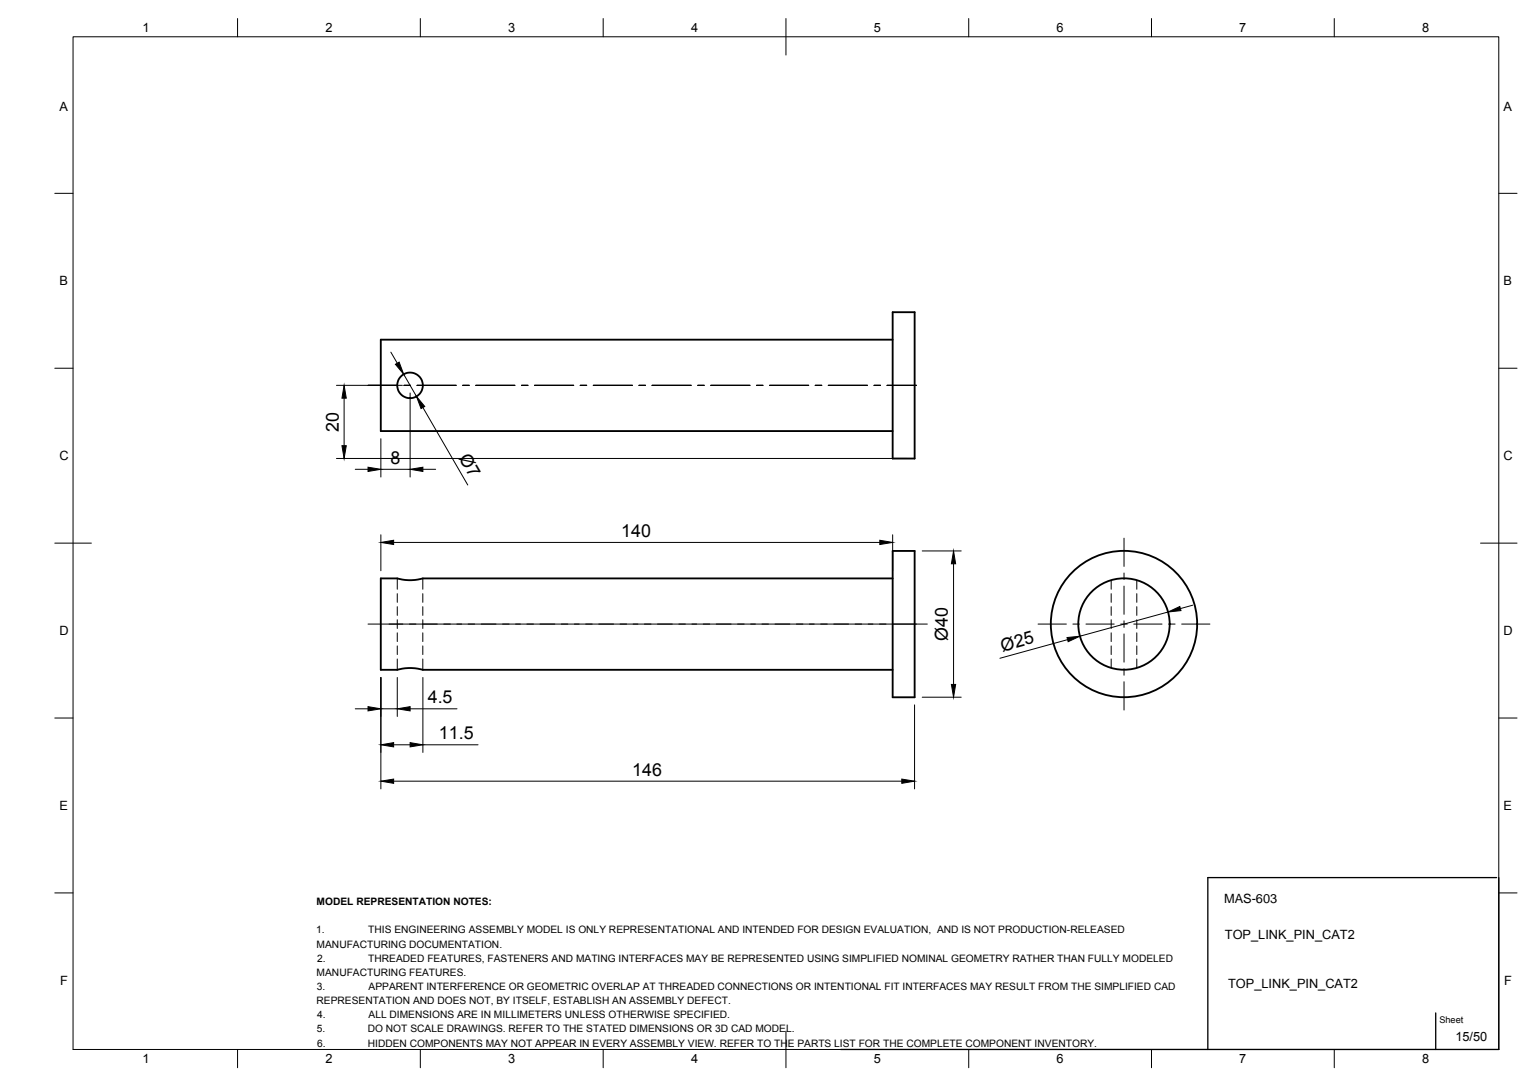
ISO-10303-21;
HEADER;
FILE_DESCRIPTION((''),'2;1');
FILE_NAME('TOP_LINK_PIN_CAT2.step','2026-10-01T22:06:14-07:00',(''),(''),'','','');
FILE_SCHEMA (('AUTOMOTIVE_DESIGN { 1 0 10303 214 3 1 1 }'));
ENDSEC;
DATA;
#10=MECHANICAL_DESIGN_GEOMETRIC_PRESENTATION_REPRESENTATION('',(#989),#50440);
#15=B_SPLINE_CURVE_WITH_KNOTS('',3,(#44967,#44968,#44969,#44970,#44971,
#44972,#44973,#44974,#44975,#44976,#44977,#44978,#44979,#44980,#44981,#44982,
#44983,#44984),.UNSPECIFIED.,.F.,.F.,(4,2,2,2,2,2,2,2,4),(0.,0.132623145855944,
0.265246291711889,0.39783980012189,0.530433308531892,0.663026816941894,
0.795620325351895,0.92824347120784,1.06086661706378),.UNSPECIFIED.) ;
#16=B_SPLINE_CURVE_WITH_KNOTS('',3,(#44985,#44986,#44987,#44988,#44989,
#44990,#44991,#44992,#44993,#44994,#44995,#44996,#44997,#44998,#44999,#45000,
#45001,#45002),.UNSPECIFIED.,.F.,.F.,(4,2,2,2,2,2,2,2,4),(1.06086661706378,
1.19348976291973,1.32611290877567,1.45870641718567,1.59129992559568,1.72389343400568,
1.85648694241568,1.98911008827162,2.12173323412757),.UNSPECIFIED.) ;
#17=B_SPLINE_CURVE_WITH_KNOTS('',3,(#45006,#45007,#45008,#45009,#45010,
#45011,#45012,#45013,#45014,#45015,#45016,#45017,#45018,#45019,#45020,#45021,
#45022,#45023),.UNSPECIFIED.,.F.,.F.,(4,2,2,2,2,2,2,2,4),(0.,0.132623145855943,
0.265246291711887,0.397839800121889,0.530433308531891,0.663026816941892,
0.795620325351894,0.928243471207838,1.06086661706378),.UNSPECIFIED.) ;
#18=B_SPLINE_CURVE_WITH_KNOTS('',3,(#45024,#45025,#45026,#45027,#45028,
#45029,#45030,#45031,#45032,#45033,#45034,#45035,#45036,#45037,#45038,#45039,
#45040,#45041),.UNSPECIFIED.,.F.,.F.,(4,2,2,2,2,2,2,2,4),(1.06086661706378,
1.19348976291973,1.32611290877567,1.45870641718567,1.59129992559567,1.72389343400568,
1.85648694241568,1.98911008827162,2.12173323412757),.UNSPECIFIED.) ;
#899=SHAPE_REPRESENTATION_RELATIONSHIP('SRR','None',#50630,#944) ;
#944=ADVANCED_BREP_SHAPE_REPRESENTATION('',(#1044),#50399) ;
#989=STYLED_ITEM('',(#50883),#1044) ;
#1044=MANIFOLD_SOLID_BREP('TOP_LINK_PIN_CAT2',#28656) ;
#1273=FACE_BOUND('',#4736,.T.) ;
#1274=FACE_BOUND('',#4740,.T.) ;
#1275=FACE_BOUND('',#4741,.T.) ;
#1929=PLANE('',#30266) ;
#1930=PLANE('',#30271) ;
#1931=PLANE('',#30274) ;
#3019=FACE_OUTER_BOUND('',#4734,.T.) ;
#3020=FACE_OUTER_BOUND('',#4735,.T.) ;
#3021=FACE_OUTER_BOUND('',#4737,.T.) ;
#3022=FACE_OUTER_BOUND('',#4738,.T.) ;
#3023=FACE_OUTER_BOUND('',#4739,.T.) ;
#3024=FACE_OUTER_BOUND('',#4742,.T.) ;
#4734=EDGE_LOOP('',(#22133,#22134,#22135,#22136,#22137,#22138)) ;
#4735=EDGE_LOOP('',(#22139)) ;
#4736=EDGE_LOOP('',(#22140)) ;
#4737=EDGE_LOOP('',(#22141,#22142,#22143,#22144)) ;
#4738=EDGE_LOOP('',(#22145)) ;
#4739=EDGE_LOOP('',(#22146,#22147,#22148,#22149)) ;
#4740=EDGE_LOOP('',(#22150,#22151)) ;
#4741=EDGE_LOOP('',(#22152,#22153)) ;
#4742=EDGE_LOOP('',(#22154)) ;
#7138=LINE('',#45004,#9610) ;
#7139=LINE('',#45049,#9611) ;
#7140=LINE('',#45055,#9612) ;
#9610=VECTOR('',#35895,0.35) ;
#9611=VECTOR('',#35904,2.) ;
#9612=VECTOR('',#35913,1.25) ;
#11002=CIRCLE('',#30267,2.) ;
#11003=CIRCLE('',#30268,1.25) ;
#11004=CIRCLE('',#30270,2.) ;
#11005=CIRCLE('',#30273,1.25) ;
#13028=VERTEX_POINT('',#44965) ;
#13029=VERTEX_POINT('',#44966) ;
#13030=VERTEX_POINT('',#45003) ;
#13031=VERTEX_POINT('',#45005) ;
#13032=VERTEX_POINT('',#45043) ;
#13033=VERTEX_POINT('',#45045) ;
#13034=VERTEX_POINT('',#45048) ;
#13035=VERTEX_POINT('',#45053) ;
#16332=EDGE_CURVE('',#13028,#13029,#15,.T.) ;
#16333=EDGE_CURVE('',#13029,#13028,#16,.T.) ;
#16334=EDGE_CURVE('',#13029,#13030,#7138,.T.) ;
#16335=EDGE_CURVE('',#13031,#13030,#17,.T.) ;
#16336=EDGE_CURVE('',#13030,#13031,#18,.T.) ;
#16337=EDGE_CURVE('',#13032,#13032,#11002,.T.) ;
#16338=EDGE_CURVE('',#13033,#13033,#11003,.T.) ;
#16339=EDGE_CURVE('',#13032,#13034,#7139,.T.) ;
#16340=EDGE_CURVE('',#13034,#13034,#11004,.T.) ;
#16341=EDGE_CURVE('',#13035,#13035,#11005,.T.) ;
#16342=EDGE_CURVE('',#13035,#13033,#7140,.T.) ;
#22133=ORIENTED_EDGE('',*,*,#16332,.F.) ;
#22134=ORIENTED_EDGE('',*,*,#16333,.F.) ;
#22135=ORIENTED_EDGE('',*,*,#16334,.T.) ;
#22136=ORIENTED_EDGE('',*,*,#16335,.F.) ;
#22137=ORIENTED_EDGE('',*,*,#16336,.F.) ;
#22138=ORIENTED_EDGE('',*,*,#16334,.F.) ;
#22139=ORIENTED_EDGE('',*,*,#16337,.T.) ;
#22140=ORIENTED_EDGE('',*,*,#16338,.T.) ;
#22141=ORIENTED_EDGE('',*,*,#16337,.F.) ;
#22142=ORIENTED_EDGE('',*,*,#16339,.T.) ;
#22143=ORIENTED_EDGE('',*,*,#16340,.F.) ;
#22144=ORIENTED_EDGE('',*,*,#16339,.F.) ;
#22145=ORIENTED_EDGE('',*,*,#16340,.T.) ;
#22146=ORIENTED_EDGE('',*,*,#16341,.F.) ;
#22147=ORIENTED_EDGE('',*,*,#16342,.T.) ;
#22148=ORIENTED_EDGE('',*,*,#16338,.F.) ;
#22149=ORIENTED_EDGE('',*,*,#16342,.F.) ;
#22150=ORIENTED_EDGE('',*,*,#16335,.T.) ;
#22151=ORIENTED_EDGE('',*,*,#16336,.T.) ;
#22152=ORIENTED_EDGE('',*,*,#16332,.T.) ;
#22153=ORIENTED_EDGE('',*,*,#16333,.T.) ;
#22154=ORIENTED_EDGE('',*,*,#16341,.T.) ;
#26779=CYLINDRICAL_SURFACE('',#30265,0.35) ;
#26780=CYLINDRICAL_SURFACE('',#30269,2.) ;
#26781=CYLINDRICAL_SURFACE('',#30272,1.25) ;
#27754=ADVANCED_FACE('',(#3019),#26779,.F.) ;
#27755=ADVANCED_FACE('',(#3020,#1273),#1929,.T.) ;
#27756=ADVANCED_FACE('',(#3021),#26780,.T.) ;
#27757=ADVANCED_FACE('',(#3022),#1930,.T.) ;
#27758=ADVANCED_FACE('',(#3023,#1274,#1275),#26781,.T.) ;
#27759=ADVANCED_FACE('',(#3024),#1931,.T.) ;
#28656=CLOSED_SHELL('',(#27754,#27755,#27756,#27757,#27758,#27759)) ;
#30264=AXIS2_PLACEMENT_3D('',#44963,#35891,#35892) ;
#30265=AXIS2_PLACEMENT_3D('',#44964,#35893,#35894) ;
#30266=AXIS2_PLACEMENT_3D('',#45042,#35896,#35897) ;
#30267=AXIS2_PLACEMENT_3D('',#45044,#35898,#35899) ;
#30268=AXIS2_PLACEMENT_3D('',#45046,#35900,#35901) ;
#30269=AXIS2_PLACEMENT_3D('',#45047,#35902,#35903) ;
#30270=AXIS2_PLACEMENT_3D('',#45050,#35905,#35906) ;
#30271=AXIS2_PLACEMENT_3D('',#45051,#35907,#35908) ;
#30272=AXIS2_PLACEMENT_3D('',#45052,#35909,#35910) ;
#30273=AXIS2_PLACEMENT_3D('',#45054,#35911,#35912) ;
#30274=AXIS2_PLACEMENT_3D('',#45056,#35914,#35915) ;
#35891=DIRECTION('axis',(0.,0.,1.)) ;
#35892=DIRECTION('refdir',(1.,0.,0.)) ;
#35893=DIRECTION('center_axis',(0.,0.,1.)) ;
#35894=DIRECTION('ref_axis',(1.,0.,0.)) ;
#35895=DIRECTION('',(0.,0.,1.)) ;
#35896=DIRECTION('center_axis',(0.,1.,0.)) ;
#35897=DIRECTION('ref_axis',(1.,0.,0.)) ;
#35898=DIRECTION('center_axis',(0.,1.,0.)) ;
#35899=DIRECTION('ref_axis',(1.,0.,0.)) ;
#35900=DIRECTION('center_axis',(0.,-1.,0.)) ;
#35901=DIRECTION('ref_axis',(1.,0.,0.)) ;
#35902=DIRECTION('center_axis',(0.,1.,0.)) ;
#35903=DIRECTION('ref_axis',(1.,0.,0.)) ;
#35904=DIRECTION('',(0.,-1.,0.)) ;
#35905=DIRECTION('center_axis',(0.,-1.,0.)) ;
#35906=DIRECTION('ref_axis',(1.,0.,0.)) ;
#35907=DIRECTION('center_axis',(0.,-1.,0.)) ;
#35908=DIRECTION('ref_axis',(-1.,0.,0.)) ;
#35909=DIRECTION('center_axis',(0.,1.,0.)) ;
#35910=DIRECTION('ref_axis',(1.,0.,0.)) ;
#35911=DIRECTION('center_axis',(0.,1.,0.)) ;
#35912=DIRECTION('ref_axis',(1.,0.,0.)) ;
#35913=DIRECTION('',(0.,-1.,0.)) ;
#35914=DIRECTION('center_axis',(0.,1.,0.)) ;
#35915=DIRECTION('ref_axis',(1.,0.,0.)) ;
#44963=CARTESIAN_POINT('',(0.,0.,0.)) ;
#44964=CARTESIAN_POINT('Origin',(0.,6.2,0.)) ;
#44965=CARTESIAN_POINT('',(0.35,6.2,-1.2)) ;
#44966=CARTESIAN_POINT('',(-0.35,6.2,-1.2)) ;
#44967=CARTESIAN_POINT('Ctrl Pts',(0.35,6.2,-1.2)) ;
#44968=CARTESIAN_POINT('Ctrl Pts',(0.35,6.24420771528532,-1.2)) ;
#44969=CARTESIAN_POINT('Ctrl Pts',(0.341116483481416,6.29118921098472,-1.20269809843758)) ;
#44970=CARTESIAN_POINT('Ctrl Pts',(0.305327067985986,6.37734520909255,-1.21227824404827)) ;
#44971=CARTESIAN_POINT('Ctrl Pts',(0.278432902947626,6.41654184388296,-1.21900443594306)) ;
#44972=CARTESIAN_POINT('Ctrl Pts',(0.216548759315801,6.47842598751478,-1.23150431818794)) ;
#44973=CARTESIAN_POINT('Ctrl Pts',(0.17734928463595,6.50532552372056,-1.23811350479585)) ;
#44974=CARTESIAN_POINT('Ctrl Pts',(0.0911830720846971,6.54111888486695,
-1.24742272978092)) ;
#44975=CARTESIAN_POINT('Ctrl Pts',(0.0441978361366672,6.55,-1.25)) ;
#44976=CARTESIAN_POINT('Ctrl Pts',(-0.0441978361366672,6.55,-1.25)) ;
#44977=CARTESIAN_POINT('Ctrl Pts',(-0.0911830720846971,6.54111888486695,
-1.24742272978092)) ;
#44978=CARTESIAN_POINT('Ctrl Pts',(-0.17734928463595,6.50532552372056,-1.23811350479585)) ;
#44979=CARTESIAN_POINT('Ctrl Pts',(-0.216548759315801,6.47842598751478,
-1.23150431818794)) ;
#44980=CARTESIAN_POINT('Ctrl Pts',(-0.278432902947626,6.41654184388296,
-1.21900443594306)) ;
#44981=CARTESIAN_POINT('Ctrl Pts',(-0.305327067985986,6.37734520909255,
-1.21227824404827)) ;
#44982=CARTESIAN_POINT('Ctrl Pts',(-0.341116483481416,6.29118921098472,
-1.20269809843758)) ;
#44983=CARTESIAN_POINT('Ctrl Pts',(-0.35,6.24420771528531,-1.2)) ;
#44984=CARTESIAN_POINT('Ctrl Pts',(-0.35,6.2,-1.2)) ;
#44985=CARTESIAN_POINT('Ctrl Pts',(-0.35,6.2,-1.2)) ;
#44986=CARTESIAN_POINT('Ctrl Pts',(-0.35,6.15579228471469,-1.2)) ;
#44987=CARTESIAN_POINT('Ctrl Pts',(-0.341116483481416,6.10881078901528,
-1.20269809843758)) ;
#44988=CARTESIAN_POINT('Ctrl Pts',(-0.305327067985986,6.02265479090746,
-1.21227824404827)) ;
#44989=CARTESIAN_POINT('Ctrl Pts',(-0.278432902947626,5.98345815611704,
-1.21900443594306)) ;
#44990=CARTESIAN_POINT('Ctrl Pts',(-0.216548759315801,5.92157401248522,
-1.23150431818794)) ;
#44991=CARTESIAN_POINT('Ctrl Pts',(-0.17734928463595,5.89467447627944,-1.23811350479585)) ;
#44992=CARTESIAN_POINT('Ctrl Pts',(-0.0911830720846975,5.85888111513305,
-1.24742272978092)) ;
#44993=CARTESIAN_POINT('Ctrl Pts',(-0.0441978361366672,5.85,-1.25)) ;
#44994=CARTESIAN_POINT('Ctrl Pts',(0.0441978361366673,5.85,-1.25)) ;
#44995=CARTESIAN_POINT('Ctrl Pts',(0.0911830720846976,5.85888111513305,
-1.24742272978092)) ;
#44996=CARTESIAN_POINT('Ctrl Pts',(0.177349284635951,5.89467447627944,-1.23811350479585)) ;
#44997=CARTESIAN_POINT('Ctrl Pts',(0.216548759315801,5.92157401248522,-1.23150431818794)) ;
#44998=CARTESIAN_POINT('Ctrl Pts',(0.278432902947626,5.98345815611704,-1.21900443594306)) ;
#44999=CARTESIAN_POINT('Ctrl Pts',(0.305327067985986,6.02265479090746,-1.21227824404827)) ;
#45000=CARTESIAN_POINT('Ctrl Pts',(0.341116483481416,6.10881078901528,-1.20269809843758)) ;
#45001=CARTESIAN_POINT('Ctrl Pts',(0.35,6.15579228471469,-1.2)) ;
#45002=CARTESIAN_POINT('Ctrl Pts',(0.35,6.2,-1.2)) ;
#45003=CARTESIAN_POINT('',(-0.35,6.2,1.2)) ;
#45004=CARTESIAN_POINT('',(-0.35,6.2,0.)) ;
#45005=CARTESIAN_POINT('',(0.35,6.2,1.2)) ;
#45006=CARTESIAN_POINT('Ctrl Pts',(0.35,6.2,1.2)) ;
#45007=CARTESIAN_POINT('Ctrl Pts',(0.35,6.15579228471469,1.2)) ;
#45008=CARTESIAN_POINT('Ctrl Pts',(0.341116483481416,6.10881078901528,1.20269809843758)) ;
#45009=CARTESIAN_POINT('Ctrl Pts',(0.305327067985986,6.02265479090746,1.21227824404827)) ;
#45010=CARTESIAN_POINT('Ctrl Pts',(0.278432902947626,5.98345815611704,1.21900443594306)) ;
#45011=CARTESIAN_POINT('Ctrl Pts',(0.216548759315801,5.92157401248522,1.23150431818794)) ;
#45012=CARTESIAN_POINT('Ctrl Pts',(0.177349284635951,5.89467447627944,1.23811350479585)) ;
#45013=CARTESIAN_POINT('Ctrl Pts',(0.0911830720846975,5.85888111513305,
1.24742272978092)) ;
#45014=CARTESIAN_POINT('Ctrl Pts',(0.0441978361366673,5.85,1.25)) ;
#45015=CARTESIAN_POINT('Ctrl Pts',(-0.0441978361366672,5.85,1.25)) ;
#45016=CARTESIAN_POINT('Ctrl Pts',(-0.0911830720846974,5.85888111513305,
1.24742272978092)) ;
#45017=CARTESIAN_POINT('Ctrl Pts',(-0.17734928463595,5.89467447627944,1.23811350479585)) ;
#45018=CARTESIAN_POINT('Ctrl Pts',(-0.216548759315801,5.92157401248522,
1.23150431818794)) ;
#45019=CARTESIAN_POINT('Ctrl Pts',(-0.278432902947626,5.98345815611704,
1.21900443594306)) ;
#45020=CARTESIAN_POINT('Ctrl Pts',(-0.305327067985986,6.02265479090746,
1.21227824404827)) ;
#45021=CARTESIAN_POINT('Ctrl Pts',(-0.341116483481416,6.10881078901528,
1.20269809843758)) ;
#45022=CARTESIAN_POINT('Ctrl Pts',(-0.35,6.15579228471469,1.2)) ;
#45023=CARTESIAN_POINT('Ctrl Pts',(-0.35,6.2,1.2)) ;
#45024=CARTESIAN_POINT('Ctrl Pts',(-0.35,6.2,1.2)) ;
#45025=CARTESIAN_POINT('Ctrl Pts',(-0.35,6.24420771528531,1.2)) ;
#45026=CARTESIAN_POINT('Ctrl Pts',(-0.341116483481416,6.29118921098472,
1.20269809843758)) ;
#45027=CARTESIAN_POINT('Ctrl Pts',(-0.305327067985986,6.37734520909255,
1.21227824404827)) ;
#45028=CARTESIAN_POINT('Ctrl Pts',(-0.278432902947626,6.41654184388296,
1.21900443594306)) ;
#45029=CARTESIAN_POINT('Ctrl Pts',(-0.216548759315801,6.47842598751478,
1.23150431818794)) ;
#45030=CARTESIAN_POINT('Ctrl Pts',(-0.177349284635951,6.50532552372056,
1.23811350479585)) ;
#45031=CARTESIAN_POINT('Ctrl Pts',(-0.0911830720846972,6.54111888486695,
1.24742272978092)) ;
#45032=CARTESIAN_POINT('Ctrl Pts',(-0.0441978361366672,6.55,1.25)) ;
#45033=CARTESIAN_POINT('Ctrl Pts',(0.0441978361366672,6.55,1.25)) ;
#45034=CARTESIAN_POINT('Ctrl Pts',(0.091183072084697,6.54111888486695,1.24742272978092)) ;
#45035=CARTESIAN_POINT('Ctrl Pts',(0.17734928463595,6.50532552372056,1.23811350479585)) ;
#45036=CARTESIAN_POINT('Ctrl Pts',(0.216548759315801,6.47842598751478,1.23150431818794)) ;
#45037=CARTESIAN_POINT('Ctrl Pts',(0.278432902947626,6.41654184388296,1.21900443594306)) ;
#45038=CARTESIAN_POINT('Ctrl Pts',(0.305327067985986,6.37734520909255,1.21227824404827)) ;
#45039=CARTESIAN_POINT('Ctrl Pts',(0.341116483481416,6.29118921098472,1.20269809843758)) ;
#45040=CARTESIAN_POINT('Ctrl Pts',(0.35,6.24420771528531,1.2)) ;
#45041=CARTESIAN_POINT('Ctrl Pts',(0.35,6.2,1.2)) ;
#45042=CARTESIAN_POINT('Origin',(0.,-7.,0.)) ;
#45043=CARTESIAN_POINT('',(-2.,-7.,2.44929359829471E-16)) ;
#45044=CARTESIAN_POINT('Origin',(0.,-7.,0.)) ;
#45045=CARTESIAN_POINT('',(-1.25,-7.,1.53080849893419E-16)) ;
#45046=CARTESIAN_POINT('Origin',(0.,-7.,0.)) ;
#45047=CARTESIAN_POINT('Origin',(0.,-7.3,0.)) ;
#45048=CARTESIAN_POINT('',(-2.,-7.6,2.44929359829471E-16)) ;
#45049=CARTESIAN_POINT('',(-2.,-7.3,2.44929359829471E-16)) ;
#45050=CARTESIAN_POINT('Origin',(0.,-7.6,0.)) ;
#45051=CARTESIAN_POINT('Origin',(0.,-7.6,0.)) ;
#45052=CARTESIAN_POINT('Origin',(0.,0.,0.)) ;
#45053=CARTESIAN_POINT('',(-1.25,7.,1.53080849893419E-16)) ;
#45054=CARTESIAN_POINT('Origin',(0.,7.,0.)) ;
#45055=CARTESIAN_POINT('',(-1.25,0.,1.53080849893419E-16)) ;
#45056=CARTESIAN_POINT('Origin',(0.,7.,0.)) ;
#50346=UNCERTAINTY_MEASURE_WITH_UNIT(LENGTH_MEASURE(0.001),#50441,
'DISTANCE_ACCURACY_VALUE',
'Maximum model space distance between geometric entities at asserted c
onnectivities') ;
#50387=UNCERTAINTY_MEASURE_WITH_UNIT(LENGTH_MEASURE(0.001),#50441,
'DISTANCE_ACCURACY_VALUE',
'Maximum model space distance between geometric entities at asserted c
onnectivities') ;
#50399=(
GEOMETRIC_REPRESENTATION_CONTEXT(3)
GLOBAL_UNCERTAINTY_ASSIGNED_CONTEXT((#50346))
GLOBAL_UNIT_ASSIGNED_CONTEXT((#50441,#50443,#50444))
REPRESENTATION_CONTEXT('','3D')
) ;
#50440=(
GEOMETRIC_REPRESENTATION_CONTEXT(3)
GLOBAL_UNCERTAINTY_ASSIGNED_CONTEXT((#50387))
GLOBAL_UNIT_ASSIGNED_CONTEXT((#50441,#50443,#50444))
REPRESENTATION_CONTEXT('','3D')
) ;
#50441=(
LENGTH_UNIT()
NAMED_UNIT(*)
SI_UNIT(.CENTI.,.METRE.)
) ;
#50443=(
NAMED_UNIT(*)
PLANE_ANGLE_UNIT()
SI_UNIT($,.RADIAN.)
) ;
#50444=(
NAMED_UNIT(*)
SI_UNIT($,.STERADIAN.)
SOLID_ANGLE_UNIT()
) ;
#50456=SHAPE_DEFINITION_REPRESENTATION(#50514,#50630) ;
#50514=PRODUCT_DEFINITION_SHAPE('',$,#50683) ;
#50630=SHAPE_REPRESENTATION('',(#30264),#50399) ;
#50671=PRODUCT_DEFINITION_CONTEXT('part definition',#50829,'design') ;
#50683=PRODUCT_DEFINITION('TOP_LINK_PIN_CAT2','TOP_LINK_PIN_CAT2',
#50735,#50671) ;
#50735=PRODUCT_DEFINITION_FORMATION('',$,#50842) ;
#50829=APPLICATION_CONTEXT(
'Core Data for Automotive Mechanical Design Process') ;
#50830=PRODUCT_CONTEXT('part definition',#50829,'mechanical') ;
#50842=PRODUCT('TOP_LINK_PIN_CAT2','TOP_LINK_PIN_CAT2',$,(#50830)) ;
#50883=PRESENTATION_STYLE_ASSIGNMENT((#50890)) ;
#50890=SURFACE_STYLE_USAGE(.BOTH.,#50897) ;
#50897=SURFACE_SIDE_STYLE('',(#50904)) ;
#50904=SURFACE_STYLE_FILL_AREA(#50911) ;
#50911=FILL_AREA_STYLE('Steel - Satin',(#50918)) ;
#50918=FILL_AREA_STYLE_COLOUR('Steel - Satin',#50925) ;
#50925=COLOUR_RGB('Steel - Satin', 0.31764706, 0.68627451, 0.89019608) ;
ENDSEC;
END-ISO-10303-21;
